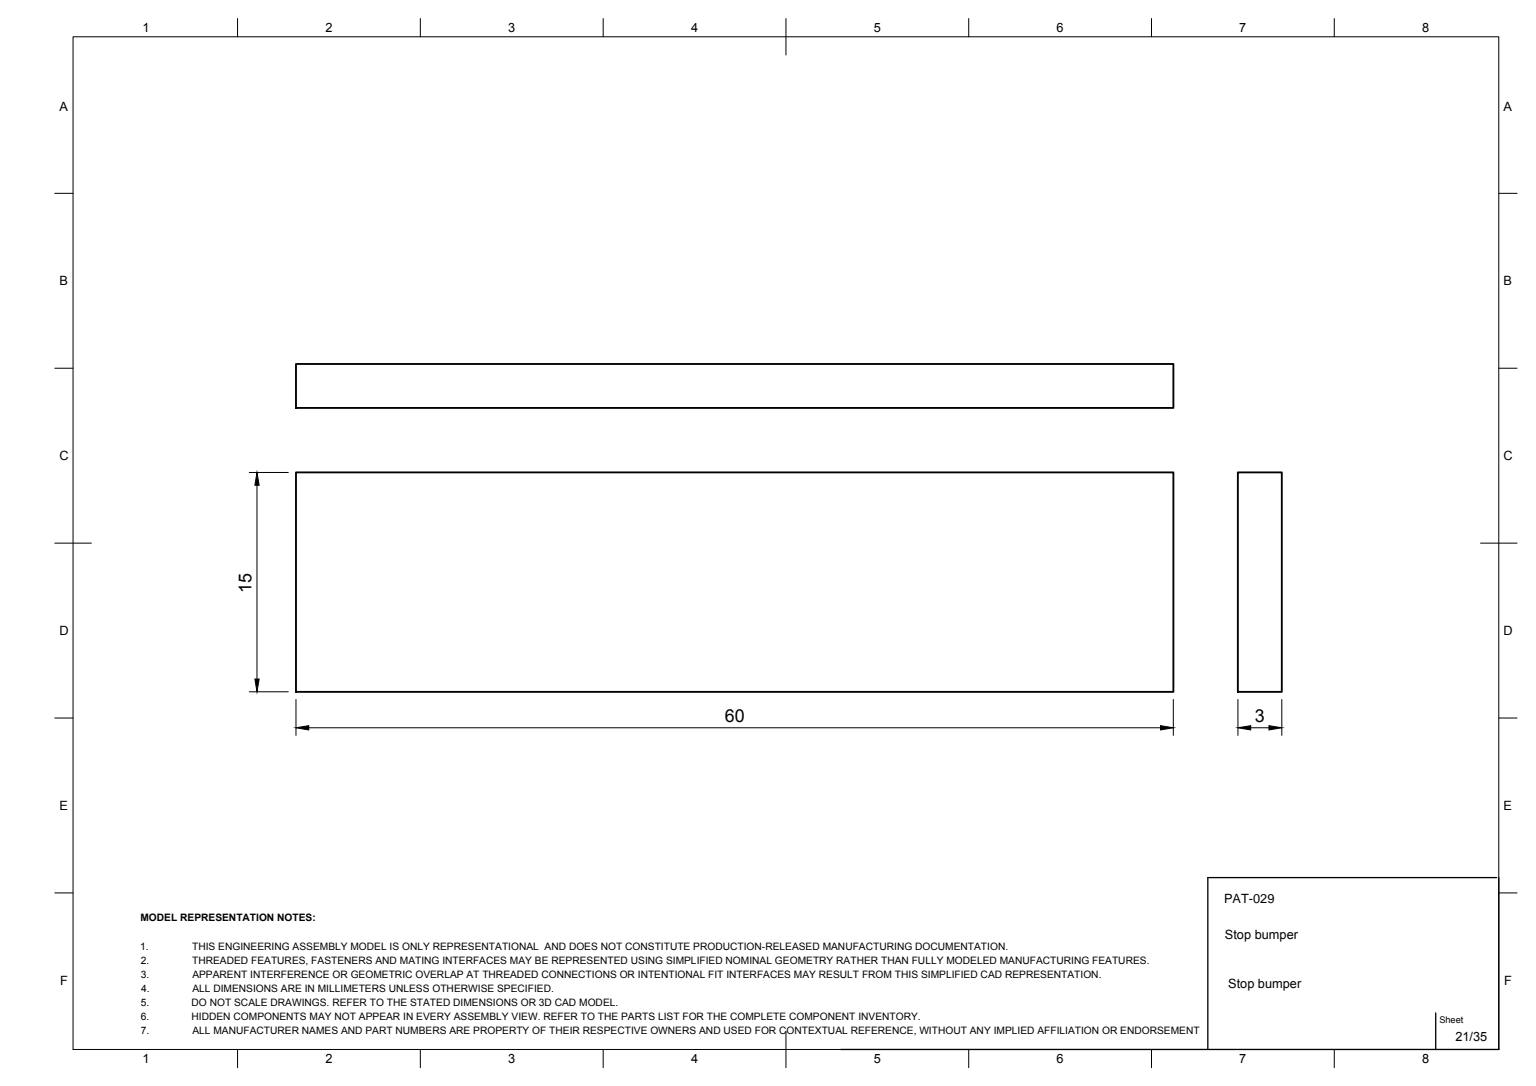
ISO-10303-21;
HEADER;
/* Generated by software containing ST-Developer
 * from STEP Tools, Inc. (www.steptools.com) 
 */

FILE_DESCRIPTION(
/* description */ ('Door-style hinge test fixture with detent'),
/* implementation_level */ '2;1');

FILE_NAME(
/* name */ 'Stop bumper.step',
/* time_stamp */ '2026-10-28T03:24:57-07:00',
/* author */ (''),
/* organization */ (''),
/* preprocessor_version */ 'ST-DEVELOPER v20.2',
/* originating_system */ 'Autodesk Translation Framework v15.17.0.0',
/* authorisation */ '');

FILE_SCHEMA (('AUTOMOTIVE_DESIGN { 1 0 10303 214 3 1 1 }'));
ENDSEC;

DATA;
#10=MECHANICAL_DESIGN_GEOMETRIC_PRESENTATION_REPRESENTATION('',(#339),#9813);
#276=SHAPE_REPRESENTATION_RELATIONSHIP('SRR','None',#9953,#307);
#307=ADVANCED_BREP_SHAPE_REPRESENTATION('',(#379),#9796);
#339=STYLED_ITEM('',(#10197),#379);
#379=MANIFOLD_SOLID_BREP('Body1',#4770);
#586=PLANE('',#5403);
#587=PLANE('',#5404);
#588=PLANE('',#5405);
#589=PLANE('',#5406);
#590=PLANE('',#5407);
#591=PLANE('',#5408);
#799=FACE_OUTER_BOUND('',#1150,.T.);
#800=FACE_OUTER_BOUND('',#1151,.T.);
#801=FACE_OUTER_BOUND('',#1152,.T.);
#802=FACE_OUTER_BOUND('',#1153,.T.);
#803=FACE_OUTER_BOUND('',#1154,.T.);
#804=FACE_OUTER_BOUND('',#1155,.T.);
#1150=EDGE_LOOP('',(#3803,#3804,#3805,#3806));
#1151=EDGE_LOOP('',(#3807,#3808,#3809,#3810));
#1152=EDGE_LOOP('',(#3811,#3812,#3813,#3814));
#1153=EDGE_LOOP('',(#3815,#3816,#3817,#3818));
#1154=EDGE_LOOP('',(#3819,#3820,#3821,#3822));
#1155=EDGE_LOOP('',(#3823,#3824,#3825,#3826));
#1520=LINE('',#8666,#1840);
#1521=LINE('',#8668,#1841);
#1522=LINE('',#8670,#1842);
#1523=LINE('',#8671,#1843);
#1524=LINE('',#8674,#1844);
#1525=LINE('',#8676,#1845);
#1526=LINE('',#8677,#1846);
#1527=LINE('',#8680,#1847);
#1528=LINE('',#8682,#1848);
#1529=LINE('',#8683,#1849);
#1530=LINE('',#8685,#1850);
#1531=LINE('',#8686,#1851);
#1840=VECTOR('',#6469,1.);
#1841=VECTOR('',#6470,1.);
#1842=VECTOR('',#6471,1.);
#1843=VECTOR('',#6472,1.);
#1844=VECTOR('',#6475,1.);
#1845=VECTOR('',#6476,1.);
#1846=VECTOR('',#6477,1.);
#1847=VECTOR('',#6480,1.);
#1848=VECTOR('',#6481,1.);
#1849=VECTOR('',#6482,1.);
#1850=VECTOR('',#6485,1.);
#1851=VECTOR('',#6486,1.);
#2421=VERTEX_POINT('',#8664);
#2422=VERTEX_POINT('',#8665);
#2423=VERTEX_POINT('',#8667);
#2424=VERTEX_POINT('',#8669);
#2425=VERTEX_POINT('',#8673);
#2426=VERTEX_POINT('',#8675);
#2427=VERTEX_POINT('',#8679);
#2428=VERTEX_POINT('',#8681);
#2918=EDGE_CURVE('',#2421,#2422,#1520,.T.);
#2919=EDGE_CURVE('',#2422,#2423,#1521,.T.);
#2920=EDGE_CURVE('',#2424,#2423,#1522,.T.);
#2921=EDGE_CURVE('',#2421,#2424,#1523,.T.);
#2922=EDGE_CURVE('',#2425,#2421,#1524,.T.);
#2923=EDGE_CURVE('',#2426,#2424,#1525,.T.);
#2924=EDGE_CURVE('',#2425,#2426,#1526,.T.);
#2925=EDGE_CURVE('',#2427,#2425,#1527,.T.);
#2926=EDGE_CURVE('',#2428,#2426,#1528,.T.);
#2927=EDGE_CURVE('',#2427,#2428,#1529,.T.);
#2928=EDGE_CURVE('',#2422,#2427,#1530,.T.);
#2929=EDGE_CURVE('',#2423,#2428,#1531,.T.);
#3803=ORIENTED_EDGE('',*,*,#2918,.T.);
#3804=ORIENTED_EDGE('',*,*,#2919,.T.);
#3805=ORIENTED_EDGE('',*,*,#2920,.F.);
#3806=ORIENTED_EDGE('',*,*,#2921,.F.);
#3807=ORIENTED_EDGE('',*,*,#2922,.T.);
#3808=ORIENTED_EDGE('',*,*,#2921,.T.);
#3809=ORIENTED_EDGE('',*,*,#2923,.F.);
#3810=ORIENTED_EDGE('',*,*,#2924,.F.);
#3811=ORIENTED_EDGE('',*,*,#2925,.T.);
#3812=ORIENTED_EDGE('',*,*,#2924,.T.);
#3813=ORIENTED_EDGE('',*,*,#2926,.F.);
#3814=ORIENTED_EDGE('',*,*,#2927,.F.);
#3815=ORIENTED_EDGE('',*,*,#2928,.T.);
#3816=ORIENTED_EDGE('',*,*,#2927,.T.);
#3817=ORIENTED_EDGE('',*,*,#2929,.F.);
#3818=ORIENTED_EDGE('',*,*,#2919,.F.);
#3819=ORIENTED_EDGE('',*,*,#2929,.T.);
#3820=ORIENTED_EDGE('',*,*,#2926,.T.);
#3821=ORIENTED_EDGE('',*,*,#2923,.T.);
#3822=ORIENTED_EDGE('',*,*,#2920,.T.);
#3823=ORIENTED_EDGE('',*,*,#2928,.F.);
#3824=ORIENTED_EDGE('',*,*,#2918,.F.);
#3825=ORIENTED_EDGE('',*,*,#2922,.F.);
#3826=ORIENTED_EDGE('',*,*,#2925,.F.);
#4604=ADVANCED_FACE('',(#799),#586,.T.);
#4605=ADVANCED_FACE('',(#800),#587,.T.);
#4606=ADVANCED_FACE('',(#801),#588,.T.);
#4607=ADVANCED_FACE('',(#802),#589,.T.);
#4608=ADVANCED_FACE('',(#803),#590,.T.);
#4609=ADVANCED_FACE('',(#804),#591,.F.);
#4770=CLOSED_SHELL('',(#4604,#4605,#4606,#4607,#4608,#4609));
#5402=AXIS2_PLACEMENT_3D('',#8662,#6465,#6466);
#5403=AXIS2_PLACEMENT_3D('',#8663,#6467,#6468);
#5404=AXIS2_PLACEMENT_3D('',#8672,#6473,#6474);
#5405=AXIS2_PLACEMENT_3D('',#8678,#6478,#6479);
#5406=AXIS2_PLACEMENT_3D('',#8684,#6483,#6484);
#5407=AXIS2_PLACEMENT_3D('',#8687,#6487,#6488);
#5408=AXIS2_PLACEMENT_3D('',#8688,#6489,#6490);
#6465=DIRECTION('axis',(0.,0.,1.));
#6466=DIRECTION('refdir',(1.,0.,0.));
#6467=DIRECTION('center_axis',(0.,1.,0.));
#6468=DIRECTION('ref_axis',(-1.,0.,0.));
#6469=DIRECTION('',(-1.,0.,0.));
#6470=DIRECTION('',(0.,0.,1.));
#6471=DIRECTION('',(-1.,0.,0.));
#6472=DIRECTION('',(0.,0.,1.));
#6473=DIRECTION('center_axis',(1.,0.,0.));
#6474=DIRECTION('ref_axis',(0.,1.,0.));
#6475=DIRECTION('',(0.,1.,0.));
#6476=DIRECTION('',(0.,1.,0.));
#6477=DIRECTION('',(0.,0.,1.));
#6478=DIRECTION('center_axis',(0.,-1.,0.));
#6479=DIRECTION('ref_axis',(1.,0.,0.));
#6480=DIRECTION('',(1.,0.,0.));
#6481=DIRECTION('',(1.,0.,0.));
#6482=DIRECTION('',(0.,0.,1.));
#6483=DIRECTION('center_axis',(-1.,0.,0.));
#6484=DIRECTION('ref_axis',(0.,-1.,0.));
#6485=DIRECTION('',(0.,-1.,0.));
#6486=DIRECTION('',(0.,-1.,0.));
#6487=DIRECTION('center_axis',(0.,0.,1.));
#6488=DIRECTION('ref_axis',(1.,0.,0.));
#6489=DIRECTION('center_axis',(0.,0.,1.));
#6490=DIRECTION('ref_axis',(1.,0.,0.));
#8662=CARTESIAN_POINT('',(0.,0.,0.));
#8663=CARTESIAN_POINT('Origin',(-0.3,11.,0.));
#8664=CARTESIAN_POINT('',(-0.3,11.,0.));
#8665=CARTESIAN_POINT('',(-0.6,11.,0.));
#8666=CARTESIAN_POINT('',(-0.3,11.,0.));
#8667=CARTESIAN_POINT('',(-0.6,11.,6.));
#8668=CARTESIAN_POINT('',(-0.6,11.,0.));
#8669=CARTESIAN_POINT('',(-0.3,11.,6.));
#8670=CARTESIAN_POINT('',(-0.3,11.,6.));
#8671=CARTESIAN_POINT('',(-0.3,11.,0.));
#8672=CARTESIAN_POINT('Origin',(-0.3,9.5,0.));
#8673=CARTESIAN_POINT('',(-0.3,9.5,0.));
#8674=CARTESIAN_POINT('',(-0.3,9.5,0.));
#8675=CARTESIAN_POINT('',(-0.3,9.5,6.));
#8676=CARTESIAN_POINT('',(-0.3,9.5,6.));
#8677=CARTESIAN_POINT('',(-0.3,9.5,0.));
#8678=CARTESIAN_POINT('Origin',(-0.6,9.5,0.));
#8679=CARTESIAN_POINT('',(-0.6,9.5,0.));
#8680=CARTESIAN_POINT('',(-0.6,9.5,0.));
#8681=CARTESIAN_POINT('',(-0.6,9.5,6.));
#8682=CARTESIAN_POINT('',(-0.6,9.5,6.));
#8683=CARTESIAN_POINT('',(-0.6,9.5,0.));
#8684=CARTESIAN_POINT('Origin',(-0.6,11.,0.));
#8685=CARTESIAN_POINT('',(-0.6,11.,0.));
#8686=CARTESIAN_POINT('',(-0.6,11.,6.));
#8687=CARTESIAN_POINT('Origin',(-0.45,10.25,6.));
#8688=CARTESIAN_POINT('Origin',(-0.45,10.25,0.));
#9760=UNCERTAINTY_MEASURE_WITH_UNIT(LENGTH_MEASURE(0.001),#9814,
'DISTANCE_ACCURACY_VALUE',
'Maximum model space distance between geometric entities at asserted c
onnectivities');
#9777=UNCERTAINTY_MEASURE_WITH_UNIT(LENGTH_MEASURE(0.001),#9814,
'DISTANCE_ACCURACY_VALUE',
'Maximum model space distance between geometric entities at asserted c
onnectivities');
#9796=(
GEOMETRIC_REPRESENTATION_CONTEXT(3)
GLOBAL_UNCERTAINTY_ASSIGNED_CONTEXT((#9760))
GLOBAL_UNIT_ASSIGNED_CONTEXT((#9814,#9816,#9817))
REPRESENTATION_CONTEXT('','3D')
);
#9813=(
GEOMETRIC_REPRESENTATION_CONTEXT(3)
GLOBAL_UNCERTAINTY_ASSIGNED_CONTEXT((#9777))
GLOBAL_UNIT_ASSIGNED_CONTEXT((#9814,#9816,#9817))
REPRESENTATION_CONTEXT('','3D')
);
#9814=(
LENGTH_UNIT()
NAMED_UNIT(*)
SI_UNIT(.CENTI.,.METRE.)
);
#9816=(
NAMED_UNIT(*)
PLANE_ANGLE_UNIT()
SI_UNIT($,.RADIAN.)
);
#9817=(
NAMED_UNIT(*)
SI_UNIT($,.STERADIAN.)
SOLID_ANGLE_UNIT()
);
#9836=SHAPE_DEFINITION_REPRESENTATION(#9871,#9953);
#9871=PRODUCT_DEFINITION_SHAPE('',$,#9989);
#9953=SHAPE_REPRESENTATION('',(#5402),#9796);
#9970=PRODUCT_DEFINITION_CONTEXT('part definition',#10077,'design');
#9989=PRODUCT_DEFINITION('Stop bumper','Stop bumper',#10024,#9970);
#10024=PRODUCT_DEFINITION_FORMATION('',$,#10097);
#10077=APPLICATION_CONTEXT(
'Core Data for Automotive Mechanical Design Process');
#10078=PRODUCT_CONTEXT('part definition',#10077,'mechanical');
#10097=PRODUCT('Stop bumper','Stop bumper','Stop bumper',(#10078));
#10191=COLOUR_RGB('Off White',0.89,0.88,0.83);
#10192=FILL_AREA_STYLE_COLOUR('',#10191);
#10193=FILL_AREA_STYLE('',(#10192));
#10194=SURFACE_STYLE_FILL_AREA(#10193);
#10195=SURFACE_SIDE_STYLE('',(#10194));
#10196=SURFACE_STYLE_USAGE(.BOTH.,#10195);
#10197=PRESENTATION_STYLE_ASSIGNMENT((#10196));
ENDSEC;
END-ISO-10303-21;
